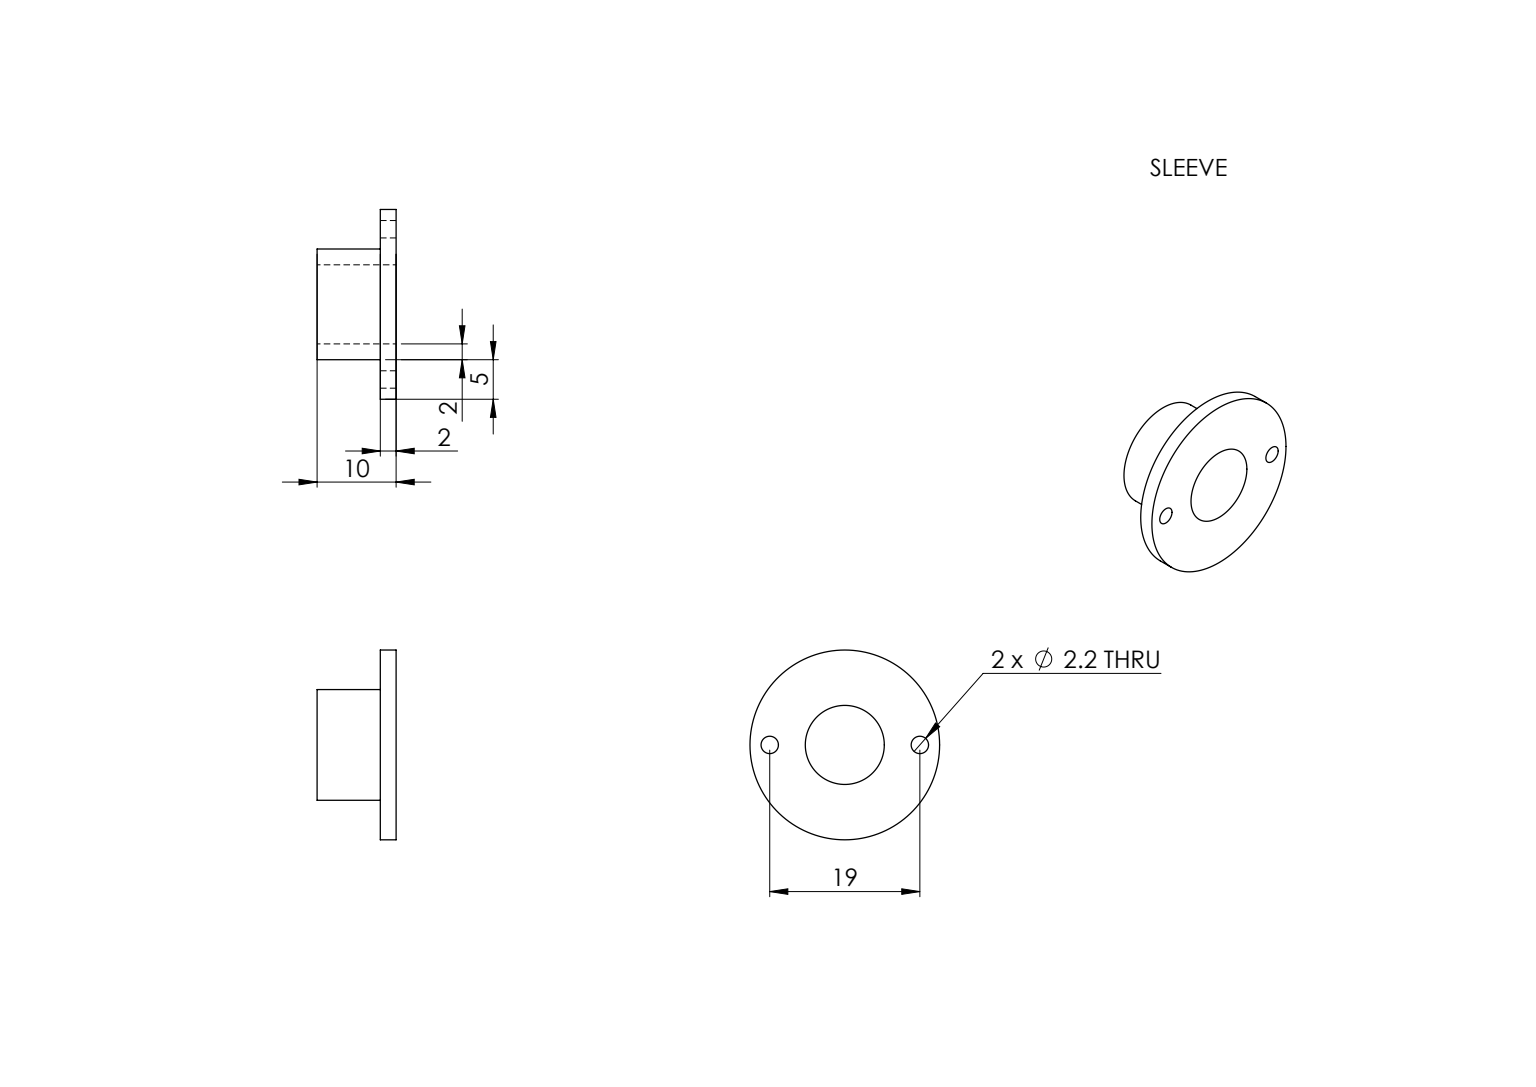
ISO-10303-21;
HEADER;
FILE_DESCRIPTION (('STEP AP214'),
    '1' );
FILE_NAME ('sleeve.step',
    '2026-10-27T14:18:53',
    ( '' ),
    ( '' ),
    'SwSTEP 2.0',
    'SolidWorks 2026',
    '' );
FILE_SCHEMA (( 'AUTOMOTIVE_DESIGN' ));
ENDSEC;

DATA;
#12=AXIS2_PLACEMENT_3D ( 'NONE', #3102, #281, #5829 ) ;
#16=AXIS2_PLACEMENT_3D ( 'NONE', #3293, #3357, #1408 ) ;
#82=DIRECTION ( 'NONE',  ( -1.000000000000000000, -0.000000000000000000, -0.000000000000000000 ) ) ;
#93=ADVANCED_FACE ( 'NONE', ( #1832 ), #5149, .T. ) ;
#96=AXIS2_PLACEMENT_3D ( 'NONE', #2644, #2066, #2156 ) ;
#106=EDGE_CURVE ( 'NONE', #5742, #4738, #1545, .T. ) ;
#119=VECTOR ( 'NONE', #946, 1000.000000000000000 ) ;
#134=CARTESIAN_POINT ( 'NONE',  ( 77.00000000000001421, 0.000000000000000000, -9.500000000000000000 ) ) ;
#163=DIRECTION ( 'NONE',  ( 1.000000000000000000, 0.000000000000000000, 0.000000000000000000 ) ) ;
#170=DIRECTION ( 'NONE',  ( 1.000000000000000000, 0.000000000000000000, 0.000000000000000000 ) ) ;
#184=EDGE_LOOP ( 'NONE', ( #1736, #1918, #2803, #4807 ) ) ;
#196=MANIFOLD_SOLID_BREP ( 'M2 Clearance Hole1', #4902 ) ;
#229=CYLINDRICAL_SURFACE ( 'NONE', #96, 5.000000000000000000 ) ;
#230=FACE_BOUND ( 'NONE', #460, .T. ) ;
#260=CARTESIAN_POINT ( 'NONE',  ( 67.00000000000001421, 6.123233995736766282E-16, 5.000000000000000000 ) ) ;
#281=DIRECTION ( 'NONE',  ( 1.000000000000000000, 0.000000000000000000, 0.000000000000000000 ) ) ;
#292=EDGE_LOOP ( 'NONE', ( #561, #1118, #3736, #5489 ) ) ;
#331=ORIENTED_EDGE ( 'NONE', *, *, #2483, .F. ) ;
#333=EDGE_CURVE ( 'NONE', #4738, #5742, #4095, .T. ) ;
#379=ORIENTED_EDGE ( 'NONE', *, *, #3057, .F. ) ;
#406=VECTOR ( 'NONE', #2782, 1000.000000000000000 ) ;
#435=AXIS2_PLACEMENT_3D ( 'NONE', #5878, #3224, #2274 ) ;
#460=EDGE_LOOP ( 'NONE', ( #331, #4146 ) ) ;
#464=DIRECTION ( 'NONE',  ( 0.000000000000000000, 0.000000000000000000, -1.000000000000000000 ) ) ;
#474=LINE ( 'NONE', #5100, #406 ) ;
#485=CARTESIAN_POINT ( 'NONE',  ( 77.00000000000001421, 0.000000000000000000, -9.500000000000000000 ) ) ;
#493=CIRCLE ( 'NONE', #4373, 1.099999999999998535 ) ;
#494=PRODUCT ( 'sleeve', 'sleeve', '', ( #2080 ) ) ;
#495=ORIENTED_EDGE ( 'NONE', *, *, #5762, .T. ) ;
#498=CIRCLE ( 'NONE', #1367, 1.099999999999998535 ) ;
#500=VERTEX_POINT ( 'NONE', #5168 ) ;
#502=VECTOR ( 'NONE', #1263, 1000.000000000000000 ) ;
#530=CARTESIAN_POINT ( 'NONE',  ( 77.00000000000001421, 0.000000000000000000, 0.000000000000000000 ) ) ;
#534=DIRECTION ( 'NONE',  ( 0.000000000000000000, 0.000000000000000000, -1.000000000000000000 ) ) ;
#545=DIRECTION ( 'NONE',  ( 0.000000000000000000, 0.000000000000000000, -1.000000000000000000 ) ) ;
#556=( LENGTH_UNIT ( ) NAMED_UNIT ( * ) SI_UNIT ( .MILLI., .METRE. ) );
#561=ORIENTED_EDGE ( 'NONE', *, *, #2602, .F. ) ;
#573=UNCERTAINTY_MEASURE_WITH_UNIT (LENGTH_MEASURE( 1.000000000000000082E-05 ), #1086, 'distance_accuracy_value', 'NONE');
#577=FACE_OUTER_BOUND ( 'NONE', #2183, .T. ) ;
#584=CARTESIAN_POINT ( 'NONE',  ( 67.00000000000001421, 0.000000000000000000, 0.000000000000000000 ) ) ;
#587=CIRCLE ( 'NONE', #1933, 1.099999999999998535 ) ;
#594=DIRECTION ( 'NONE',  ( 1.000000000000000000, -0.000000000000000000, -0.000000000000000000 ) ) ;
#597=AXIS2_PLACEMENT_3D ( 'NONE', #715, #5362, #4077 ) ;
#607=ORIENTED_EDGE ( 'NONE', *, *, #3154, .F. ) ;
#617=ADVANCED_FACE ( 'NONE', ( #2607 ), #229, .F. ) ;
#653=FACE_OUTER_BOUND ( 'NONE', #742, .T. ) ;
#661=DIRECTION ( 'NONE',  ( 1.000000000000000000, -0.000000000000000000, -0.000000000000000000 ) ) ;
#667=DIRECTION ( 'NONE',  ( 1.000000000000000000, 0.000000000000000000, 0.000000000000000000 ) ) ;
#698=VERTEX_POINT ( 'NONE', #4958 ) ;
#707=PLANE ( 'NONE',  #3487 ) ;
#715=CARTESIAN_POINT ( 'NONE',  ( 75.00000000000001421, 0.000000000000000000, 0.000000000000000000 ) ) ;
#742=EDGE_LOOP ( 'NONE', ( #3170, #5345, #1739, #1388 ) ) ;
#768=ORIENTED_EDGE ( 'NONE', *, *, #864, .F. ) ;
#793=EDGE_CURVE ( 'NONE', #853, #1083, #1370, .T. ) ;
#836=ORIENTED_EDGE ( 'NONE', *, *, #106, .F. ) ;
#853=VERTEX_POINT ( 'NONE', #1421 ) ;
#864=EDGE_CURVE ( 'NONE', #1686, #2079, #5088, .T. ) ;
#865=CIRCLE ( 'NONE', #5519, 7.000000000000000000 ) ;
#871=CIRCLE ( 'NONE', #1922, 5.000000000000000000 ) ;
#885=ORIENTED_EDGE ( 'NONE', *, *, #4953, .F. ) ;
#912=DIRECTION ( 'NONE',  ( 0.000000000000000000, 0.000000000000000000, -1.000000000000000000 ) ) ;
#940=DIRECTION ( 'NONE',  ( 1.000000000000000000, -0.000000000000000000, -0.000000000000000000 ) ) ;
#945=ADVANCED_FACE ( 'NONE', ( #1482 ), #1994, .F. ) ;
#946=DIRECTION ( 'NONE',  ( -1.000000000000000000, -0.000000000000000000, -0.000000000000000000 ) ) ;
#952=DIRECTION ( 'NONE',  ( 1.000000000000000000, 0.000000000000000000, 0.000000000000000000 ) ) ;
#986=CARTESIAN_POINT ( 'NONE',  ( 77.00000000000001421, 0.000000000000000000, 9.500000000000000000 ) ) ;
#1007=DIRECTION ( 'NONE',  ( 0.000000000000000000, 0.000000000000000000, -1.000000000000000000 ) ) ;
#1014=DIRECTION ( 'NONE',  ( 0.000000000000000000, 0.000000000000000000, -1.000000000000000000 ) ) ;
#1020=DIRECTION ( 'NONE',  ( 1.000000000000000000, 0.000000000000000000, 0.000000000000000000 ) ) ;
#1025=ORIENTED_EDGE ( 'NONE', *, *, #3057, .T. ) ;
#1033=VERTEX_POINT ( 'NONE', #5730 ) ;
#1039=CARTESIAN_POINT ( 'NONE',  ( 67.00000000000001421, 0.000000000000000000, -7.000000000000000000 ) ) ;
#1051=UNCERTAINTY_MEASURE_WITH_UNIT (LENGTH_MEASURE( 1.000000000000000082E-05 ), #556, 'distance_accuracy_value', 'NONE');
#1066=ORIENTED_EDGE ( 'NONE', *, *, #3945, .F. ) ;
#1075=CARTESIAN_POINT ( 'NONE',  ( 77.00000000000001421, 6.123233995736766282E-16, 5.000000000000000000 ) ) ;
#1079=VECTOR ( 'NONE', #4669, 1000.000000000000000 ) ;
#1083=VERTEX_POINT ( 'NONE', #2974 ) ;
#1086=( LENGTH_UNIT ( ) NAMED_UNIT ( * ) SI_UNIT ( .MILLI., .METRE. ) );
#1096=ORIENTED_EDGE ( 'NONE', *, *, #4928, .T. ) ;
#1097=EDGE_CURVE ( 'NONE', #698, #853, #5401, .T. ) ;
#1107=CARTESIAN_POINT ( 'NONE',  ( 67.00000000000001421, 0.000000000000000000, 0.000000000000000000 ) ) ;
#1118=ORIENTED_EDGE ( 'NONE', *, *, #4148, .T. ) ;
#1122=FACE_BOUND ( 'NONE', #4862, .T. ) ;
#1132=EDGE_LOOP ( 'NONE', ( #2391, #4516, #2697, #3573 ) ) ;
#1153=AXIS2_PLACEMENT_3D ( 'NONE', #1244, #5435, #4903 ) ;
#1174=EDGE_CURVE ( 'NONE', #3739, #3914, #1198, .T. ) ;
#1198=CIRCLE ( 'NONE', #435, 7.000000000000000000 ) ;
#1244=CARTESIAN_POINT ( 'NONE',  ( 77.00000000000001421, 0.000000000000000000, 0.000000000000000000 ) ) ;
#1247=ORIENTED_EDGE ( 'NONE', *, *, #2767, .F. ) ;
#1263=DIRECTION ( 'NONE',  ( 1.000000000000000000, -0.000000000000000000, -0.000000000000000000 ) ) ;
#1278=AXIS2_PLACEMENT_3D ( 'NONE', #5592, #2758, #4614 ) ;
#1300=ORIENTED_EDGE ( 'NONE', *, *, #2092, .T. ) ;
#1316=ORIENTED_EDGE ( 'NONE', *, *, #4317, .F. ) ;
#1328=LINE ( 'NONE', #3553, #3131 ) ;
#1351=CYLINDRICAL_SURFACE ( 'NONE', #1278, 1.099999999999998535 ) ;
#1359=PLANE ( 'NONE',  #4979 ) ;
#1367=AXIS2_PLACEMENT_3D ( 'NONE', #2010, #5780, #3474 ) ;
#1370=CIRCLE ( 'NONE', #3703, 1.099999999999998535 ) ;
#1371=FACE_BOUND ( 'NONE', #2481, .T. ) ;
#1388=ORIENTED_EDGE ( 'NONE', *, *, #793, .T. ) ;
#1396=ADVANCED_FACE ( 'NONE', ( #3274, #4676 ), #4731, .F. ) ;
#1408=DIRECTION ( 'NONE',  ( 0.000000000000000000, 0.000000000000000000, -1.000000000000000000 ) ) ;
#1421=CARTESIAN_POINT ( 'NONE',  ( 77.00000000000001421, 0.000000000000000000, -10.59999999999999787 ) ) ;
#1447=CARTESIAN_POINT ( 'NONE',  ( 75.00000000000001421, 0.000000000000000000, 9.500000000000000000 ) ) ;
#1453=EDGE_LOOP ( 'NONE', ( #836, #4145 ) ) ;
#1479=DIRECTION ( 'NONE',  ( 1.000000000000000000, 0.000000000000000000, 0.000000000000000000 ) ) ;
#1482=FACE_OUTER_BOUND ( 'NONE', #3024, .T. ) ;
#1487=CARTESIAN_POINT ( 'NONE',  ( 77.00000000000001421, 0.000000000000000000, 8.400000000000000355 ) ) ;
#1491=CARTESIAN_POINT ( 'NONE',  ( 77.00000000000001421, 0.000000000000000000, 0.000000000000000000 ) ) ;
#1496=CARTESIAN_POINT ( 'NONE',  ( 77.00000000000001421, 1.347111479062087271E-16, 10.59999999999999787 ) ) ;
#1509=EDGE_LOOP ( 'NONE', ( #4744, #2585 ) ) ;
#1524=VERTEX_POINT ( 'NONE', #1075 ) ;
#1544=ORIENTED_EDGE ( 'NONE', *, *, #1174, .T. ) ;
#1545=CIRCLE ( 'NONE', #4752, 12.00000000000000000 ) ;
#1554=CIRCLE ( 'NONE', #16, 5.000000000000000000 ) ;
#1566=CIRCLE ( 'NONE', #597, 7.000000000000000000 ) ;
#1596=ORIENTED_EDGE ( 'NONE', *, *, #2092, .F. ) ;
#1605=FILL_AREA_STYLE ('',( #2060 ) ) ;
#1610=EDGE_CURVE ( 'NONE', #3914, #3739, #4338, .T. ) ;
#1613=AXIS2_PLACEMENT_3D ( 'NONE', #2411, #1020, #5661 ) ;
#1621=DIRECTION ( 'NONE',  ( 1.000000000000000000, 0.000000000000000000, 0.000000000000000000 ) ) ;
#1625=CARTESIAN_POINT ( 'NONE',  ( 67.00000000000001421, 0.000000000000000000, -5.000000000000000000 ) ) ;
#1637=SURFACE_STYLE_USAGE ( .BOTH. , #5312 ) ;
#1686=VERTEX_POINT ( 'NONE', #3155 ) ;
#1700=CARTESIAN_POINT ( 'NONE',  ( 75.00000000000001421, 0.000000000000000000, 0.000000000000000000 ) ) ;
#1701=PRODUCT_DEFINITION_SHAPE ( 'NONE', 'NONE',  #2570 ) ;
#1726=DIRECTION ( 'NONE',  ( 1.000000000000000000, 0.000000000000000000, 0.000000000000000000 ) ) ;
#1736=ORIENTED_EDGE ( 'NONE', *, *, #2058, .F. ) ;
#1739=ORIENTED_EDGE ( 'NONE', *, *, #1097, .T. ) ;
#1745=AXIS2_PLACEMENT_3D ( 'NONE', #530, #82, #5327 ) ;
#1771=DIRECTION ( 'NONE',  ( 0.000000000000000000, 0.000000000000000000, -1.000000000000000000 ) ) ;
#1804=CARTESIAN_POINT ( 'NONE',  ( 75.00000000000001421, 0.000000000000000000, 0.000000000000000000 ) ) ;
#1810=CARTESIAN_POINT ( 'NONE',  ( 75.00000000000001421, 1.469576158976823947E-15, -12.00000000000000000 ) ) ;
#1813=VERTEX_POINT ( 'NONE', #1496 ) ;
#1832=FACE_OUTER_BOUND ( 'NONE', #292, .T. ) ;
#1833=AXIS2_PLACEMENT_3D ( 'NONE', #3894, #1621, #3443 ) ;
#1839=DIRECTION ( 'NONE',  ( 1.000000000000000000, -0.000000000000000000, -0.000000000000000000 ) ) ;
#1889=LINE ( 'NONE', #3356, #3200 ) ;
#1897=EDGE_CURVE ( 'NONE', #500, #1083, #1889, .T. ) ;
#1904=CARTESIAN_POINT ( 'NONE',  ( 67.00000000000001421, 0.000000000000000000, 0.000000000000000000 ) ) ;
#1913=( NAMED_UNIT ( * ) SI_UNIT ( $, .STERADIAN. ) SOLID_ANGLE_UNIT ( ) );
#1918=ORIENTED_EDGE ( 'NONE', *, *, #2276, .F. ) ;
#1922=AXIS2_PLACEMENT_3D ( 'NONE', #2652, #2830, #464 ) ;
#1933=AXIS2_PLACEMENT_3D ( 'NONE', #986, #2808, #4699 ) ;
#1942=ORIENTED_EDGE ( 'NONE', *, *, #2000, .T. ) ;
#1966=ORIENTED_EDGE ( 'NONE', *, *, #1097, .F. ) ;
#1978=CARTESIAN_POINT ( 'NONE',  ( 75.00000000000001421, 0.000000000000000000, 0.000000000000000000 ) ) ;
#1988=DIRECTION ( 'NONE',  ( 1.000000000000000000, 0.000000000000000000, 0.000000000000000000 ) ) ;
#1990=CARTESIAN_POINT ( 'NONE',  ( 77.00000000000001421, 0.000000000000000000, 9.500000000000000000 ) ) ;
#1994=CYLINDRICAL_SURFACE ( 'NONE', #5653, 5.000000000000000000 ) ;
#1995=ORIENTED_EDGE ( 'NONE', *, *, #2425, .T. ) ;
#2000=EDGE_CURVE ( 'NONE', #1524, #3408, #2315, .T. ) ;
#2010=CARTESIAN_POINT ( 'NONE',  ( 75.00000000000001421, 0.000000000000000000, -9.500000000000000000 ) ) ;
#2026=UNCERTAINTY_MEASURE_WITH_UNIT (LENGTH_MEASURE( 1.000000000000000082E-05 ), #2116, 'distance_accuracy_value', 'NONE');
#2058=EDGE_CURVE ( 'NONE', #5304, #1524, #2557, .T. ) ;
#2060=FILL_AREA_STYLE_COLOUR ( '', #2747 ) ;
#2066=DIRECTION ( 'NONE',  ( 1.000000000000000000, 0.000000000000000000, 0.000000000000000000 ) ) ;
#2079=VERTEX_POINT ( 'NONE', #5745 ) ;
#2080=PRODUCT_CONTEXT ( 'NONE', #5443, 'mechanical' ) ;
#2089=ORIENTED_EDGE ( 'NONE', *, *, #1610, .T. ) ;
#2092=EDGE_CURVE ( 'NONE', #2669, #4799, #865, .T. ) ;
#2098=EDGE_LOOP ( 'NONE', ( #3653, #1247, #495, #4762 ) ) ;
#2116=( LENGTH_UNIT ( ) NAMED_UNIT ( * ) SI_UNIT ( .MILLI., .METRE. ) );
#2123=VECTOR ( 'NONE', #170, 1000.000000000000000 ) ;
#2127=ORIENTED_EDGE ( 'NONE', *, *, #3252, .F. ) ;
#2135=AXIS2_PLACEMENT_3D ( 'NONE', #3768, #952, #1014 ) ;
#2156=DIRECTION ( 'NONE',  ( 0.000000000000000000, 0.000000000000000000, -1.000000000000000000 ) ) ;
#2164=PRODUCT_DEFINITION_FORMATION_WITH_SPECIFIED_SOURCE ( 'ANY', '', #494, .NOT_KNOWN. ) ;
#2183=EDGE_LOOP ( 'NONE', ( #3761, #5439, #4702, #1966 ) ) ;
#2227=CIRCLE ( 'NONE', #2423, 12.00000000000000000 ) ;
#2232=CARTESIAN_POINT ( 'NONE',  ( 67.00000000000001421, 0.000000000000000000, 0.000000000000000000 ) ) ;
#2237=CIRCLE ( 'NONE', #3780, 1.099999999999998535 ) ;
#2251=ORIENTED_EDGE ( 'NONE', *, *, #5010, .F. ) ;
#2257=MECHANICAL_DESIGN_GEOMETRIC_PRESENTATION_REPRESENTATION('',(#4595),#3711);
#2274=DIRECTION ( 'NONE',  ( 0.000000000000000000, 0.000000000000000000, -1.000000000000000000 ) ) ;
#2276=EDGE_CURVE ( 'NONE', #3852, #5304, #871, .T. ) ;
#2315=CIRCLE ( 'NONE', #1833, 5.000000000000000000 ) ;
#2321=AXIS2_PLACEMENT_3D ( 'NONE', #4119, #2350, #4083 ) ;
#2322=CARTESIAN_POINT ( 'NONE',  ( 77.00000000000001421, 0.000000000000000000, -9.500000000000000000 ) ) ;
#2323=CIRCLE ( 'NONE', #12, 5.000000000000000000 ) ;
#2330=DIRECTION ( 'NONE',  ( 1.000000000000000000, -0.000000000000000000, -0.000000000000000000 ) ) ;
#2338=CARTESIAN_POINT ( 'NONE',  ( 75.00000000000001421, 0.000000000000000000, 0.000000000000000000 ) ) ;
#2344=ADVANCED_FACE ( 'NONE', ( #1371, #1122, #2920, #230 ), #707, .T. ) ;
#2350=DIRECTION ( 'NONE',  ( -1.000000000000000000, -0.000000000000000000, -0.000000000000000000 ) ) ;
#2362=VECTOR ( 'NONE', #4861, 1000.000000000000000 ) ;
#2366=DIRECTION ( 'NONE',  ( 0.000000000000000000, 0.000000000000000000, -1.000000000000000000 ) ) ;
#2391=ORIENTED_EDGE ( 'NONE', *, *, #3208, .F. ) ;
#2411=CARTESIAN_POINT ( 'NONE',  ( 67.00000000000001421, 0.000000000000000000, 0.000000000000000000 ) ) ;
#2423=AXIS2_PLACEMENT_3D ( 'NONE', #4705, #1988, #2874 ) ;
#2425=EDGE_CURVE ( 'NONE', #500, #698, #2610, .T. ) ;
#2429=CYLINDRICAL_SURFACE ( 'NONE', #4096, 1.099999999999998535 ) ;
#2438=AXIS2_PLACEMENT_3D ( 'NONE', #584, #5675, #1007 ) ;
#2462=CARTESIAN_POINT ( 'NONE',  ( 75.00000000000001421, 0.000000000000000000, -9.500000000000000000 ) ) ;
#2463=ORIENTED_EDGE ( 'NONE', *, *, #4160, .F. ) ;
#2481=EDGE_LOOP ( 'NONE', ( #379, #2127 ) ) ;
#2482=AXIS2_PLACEMENT_3D ( 'NONE', #1107, #5754, #4337 ) ;
#2483=EDGE_CURVE ( 'NONE', #3408, #1524, #2323, .T. ) ;
#2513=MECHANICAL_DESIGN_GEOMETRIC_PRESENTATION_REPRESENTATION('',(#5058),#3689);
#2552=DIRECTION ( 'NONE',  ( 0.000000000000000000, 0.000000000000000000, -1.000000000000000000 ) ) ;
#2557=LINE ( 'NONE', #260, #2123 ) ;
#2570=PRODUCT_DEFINITION ( 'UNKNOWN', '', #2164, #5792 ) ;
#2574=( NAMED_UNIT ( * ) SI_UNIT ( $, .STERADIAN. ) SOLID_ANGLE_UNIT ( ) );
#2585=ORIENTED_EDGE ( 'NONE', *, *, #1610, .F. ) ;
#2596=CARTESIAN_POINT ( 'NONE',  ( 77.00000000000001421, 0.000000000000000000, 8.400000000000000355 ) ) ;
#2602=EDGE_CURVE ( 'NONE', #5213, #1033, #2614, .T. ) ;
#2607=FACE_OUTER_BOUND ( 'NONE', #184, .T. ) ;
#2610=CIRCLE ( 'NONE', #4169, 1.099999999999998535 ) ;
#2614=CIRCLE ( 'NONE', #1153, 12.00000000000000000 ) ;
#2644=CARTESIAN_POINT ( 'NONE',  ( 67.00000000000001421, 0.000000000000000000, 0.000000000000000000 ) ) ;
#2647=( GEOMETRIC_REPRESENTATION_CONTEXT ( 3 ) GLOBAL_UNCERTAINTY_ASSIGNED_CONTEXT ( ( #2026 ) ) GLOBAL_UNIT_ASSIGNED_CONTEXT ( ( #2116, #5374, #4344 ) ) REPRESENTATION_CONTEXT ( 'NONE', 'WORKASPACE' ) );
#2652=CARTESIAN_POINT ( 'NONE',  ( 67.00000000000001421, 0.000000000000000000, 0.000000000000000000 ) ) ;
#2669=VERTEX_POINT ( 'NONE', #3811 ) ;
#2670=DIRECTION ( 'NONE',  ( 1.000000000000000000, -0.000000000000000000, -0.000000000000000000 ) ) ;
#2697=ORIENTED_EDGE ( 'NONE', *, *, #3252, .T. ) ;
#2703=ORIENTED_EDGE ( 'NONE', *, *, #2602, .T. ) ;
#2747=COLOUR_RGB ( '',0.8941176470588234615, 0.8941176470588234615, 0.8941176470588234615 ) ;
#2758=DIRECTION ( 'NONE',  ( 1.000000000000000000, -0.000000000000000000, -0.000000000000000000 ) ) ;
#2767=EDGE_CURVE ( 'NONE', #1033, #5213, #2227, .T. ) ;
#2782=DIRECTION ( 'NONE',  ( 1.000000000000000000, 0.000000000000000000, 0.000000000000000000 ) ) ;
#2795=DIRECTION ( 'NONE',  ( 0.000000000000000000, 0.000000000000000000, -1.000000000000000000 ) ) ;
#2801=LINE ( 'NONE', #4144, #3506 ) ;
#2803=ORIENTED_EDGE ( 'NONE', *, *, #5010, .T. ) ;
#2808=DIRECTION ( 'NONE',  ( 1.000000000000000000, -0.000000000000000000, -0.000000000000000000 ) ) ;
#2830=DIRECTION ( 'NONE',  ( 1.000000000000000000, 0.000000000000000000, 0.000000000000000000 ) ) ;
#2840=ADVANCED_FACE ( 'NONE', ( #577 ), #2429, .F. ) ;
#2874=DIRECTION ( 'NONE',  ( 0.000000000000000000, 0.000000000000000000, -1.000000000000000000 ) ) ;
#2907=DIRECTION ( 'NONE',  ( 0.000000000000000000, 0.000000000000000000, -1.000000000000000000 ) ) ;
#2920=FACE_OUTER_BOUND ( 'NONE', #5697, .T. ) ;
#2941=FACE_OUTER_BOUND ( 'NONE', #3622, .T. ) ;
#2974=CARTESIAN_POINT ( 'NONE',  ( 77.00000000000001421, 1.347111479062087271E-16, -8.400000000000000355 ) ) ;
#3024=EDGE_LOOP ( 'NONE', ( #607, #3147, #1942, #2251 ) ) ;
#3037=( NAMED_UNIT ( * ) PLANE_ANGLE_UNIT ( ) SI_UNIT ( $, .RADIAN. ) );
#3057=EDGE_CURVE ( 'NONE', #5651, #1813, #493, .T. ) ;
#3062=DIRECTION ( 'NONE',  ( 0.000000000000000000, 0.000000000000000000, -1.000000000000000000 ) ) ;
#3102=CARTESIAN_POINT ( 'NONE',  ( 77.00000000000001421, 0.000000000000000000, 0.000000000000000000 ) ) ;
#3105=ORIENTED_EDGE ( 'NONE', *, *, #3154, .T. ) ;
#3122=FACE_OUTER_BOUND ( 'NONE', #4657, .T. ) ;
#3131=VECTOR ( 'NONE', #2670, 1000.000000000000000 ) ;
#3133=DIRECTION ( 'NONE',  ( 0.000000000000000000, 0.000000000000000000, -1.000000000000000000 ) ) ;
#3147=ORIENTED_EDGE ( 'NONE', *, *, #2058, .T. ) ;
#3154=EDGE_CURVE ( 'NONE', #5304, #3852, #1554, .T. ) ;
#3155=CARTESIAN_POINT ( 'NONE',  ( 75.00000000000001421, 0.000000000000000000, 8.400000000000000355 ) ) ;
#3163=FACE_BOUND ( 'NONE', #5469, .T. ) ;
#3170=ORIENTED_EDGE ( 'NONE', *, *, #1897, .F. ) ;
#3200=VECTOR ( 'NONE', #4178, 1000.000000000000000 ) ;
#3208=EDGE_CURVE ( 'NONE', #2079, #1686, #3690, .T. ) ;
#3224=DIRECTION ( 'NONE',  ( 1.000000000000000000, 0.000000000000000000, 0.000000000000000000 ) ) ;
#3252=EDGE_CURVE ( 'NONE', #1813, #5651, #587, .T. ) ;
#3254=SHAPE_REPRESENTATION ( 'sleeve', ( #5080 ), #2647 ) ;
#3259=ADVANCED_FACE ( 'NONE', ( #4213 ), #5591, .T. ) ;
#3274=FACE_BOUND ( 'NONE', #4241, .T. ) ;
#3293=CARTESIAN_POINT ( 'NONE',  ( 67.00000000000001421, 0.000000000000000000, 0.000000000000000000 ) ) ;
#3297=CARTESIAN_POINT ( 'NONE',  ( 67.00000000000001421, 0.000000000000000000, -5.000000000000000000 ) ) ;
#3299=ORIENTED_EDGE ( 'NONE', *, *, #3945, .T. ) ;
#3308=DIRECTION ( 'NONE',  ( 1.000000000000000000, 0.000000000000000000, 0.000000000000000000 ) ) ;
#3331=LINE ( 'NONE', #5179, #1079 ) ;
#3348=CYLINDRICAL_SURFACE ( 'NONE', #2438, 7.000000000000000000 ) ;
#3356=CARTESIAN_POINT ( 'NONE',  ( 77.00000000000001421, 1.347111479062087271E-16, -8.400000000000000355 ) ) ;
#3357=DIRECTION ( 'NONE',  ( 1.000000000000000000, 0.000000000000000000, 0.000000000000000000 ) ) ;
#3369=DIRECTION ( 'NONE',  ( 1.000000000000000000, 0.000000000000000000, 0.000000000000000000 ) ) ;
#3408=VERTEX_POINT ( 'NONE', #4539 ) ;
#3413=DIRECTION ( 'NONE',  ( 1.000000000000000000, 0.000000000000000000, 0.000000000000000000 ) ) ;
#3443=DIRECTION ( 'NONE',  ( 0.000000000000000000, 0.000000000000000000, -1.000000000000000000 ) ) ;
#3458=SURFACE_STYLE_FILL_AREA ( #1605 ) ;
#3474=DIRECTION ( 'NONE',  ( 0.000000000000000000, 0.000000000000000000, -1.000000000000000000 ) ) ;
#3487=AXIS2_PLACEMENT_3D ( 'NONE', #1491, #3917, #2552 ) ;
#3506=VECTOR ( 'NONE', #1479, 1000.000000000000000 ) ;
#3527=CARTESIAN_POINT ( 'NONE',  ( 0.000000000000000000, 0.000000000000000000, 0.000000000000000000 ) ) ;
#3540=CARTESIAN_POINT ( 'NONE',  ( 67.00000000000001421, 6.123233995736766282E-16, 5.000000000000000000 ) ) ;
#3547=DIRECTION ( 'NONE',  ( 1.000000000000000000, 0.000000000000000000, 0.000000000000000000 ) ) ;
#3553=CARTESIAN_POINT ( 'NONE',  ( 77.00000000000001421, 1.347111479062087271E-16, 10.59999999999999787 ) ) ;
#3573=ORIENTED_EDGE ( 'NONE', *, *, #5640, .F. ) ;
#3579=APPLICATION_CONTEXT ( 'automotive_design' ) ;
#3622=EDGE_LOOP ( 'NONE', ( #1316, #768, #4153, #1025 ) ) ;
#3653=ORIENTED_EDGE ( 'NONE', *, *, #4148, .F. ) ;
#3689=( GEOMETRIC_REPRESENTATION_CONTEXT ( 3 ) GLOBAL_UNCERTAINTY_ASSIGNED_CONTEXT ( ( #1051 ) ) GLOBAL_UNIT_ASSIGNED_CONTEXT ( ( #556, #4235, #1913 ) ) REPRESENTATION_CONTEXT ( 'NONE', 'WORKASPACE' ) );
#3690=CIRCLE ( 'NONE', #2135, 1.099999999999998535 ) ;
#3703=AXIS2_PLACEMENT_3D ( 'NONE', #485, #2330, #912 ) ;
#3711=( GEOMETRIC_REPRESENTATION_CONTEXT ( 3 ) GLOBAL_UNCERTAINTY_ASSIGNED_CONTEXT ( ( #573 ) ) GLOBAL_UNIT_ASSIGNED_CONTEXT ( ( #1086, #3037, #2574 ) ) REPRESENTATION_CONTEXT ( 'NONE', 'WORKASPACE' ) );
#3716=AXIS2_PLACEMENT_3D ( 'NONE', #1447, #3369, #545 ) ;
#3736=ORIENTED_EDGE ( 'NONE', *, *, #333, .T. ) ;
#3739=VERTEX_POINT ( 'NONE', #1039 ) ;
#3761=ORIENTED_EDGE ( 'NONE', *, *, #2425, .F. ) ;
#3768=CARTESIAN_POINT ( 'NONE',  ( 75.00000000000001421, 0.000000000000000000, 9.500000000000000000 ) ) ;
#3780=AXIS2_PLACEMENT_3D ( 'NONE', #2322, #1839, #534 ) ;
#3811=CARTESIAN_POINT ( 'NONE',  ( 75.00000000000001421, 8.572527594031473190E-16, 7.000000000000000000 ) ) ;
#3832=DIRECTION ( 'NONE',  ( 0.000000000000000000, 0.000000000000000000, -1.000000000000000000 ) ) ;
#3842=ORIENTED_EDGE ( 'NONE', *, *, #793, .F. ) ;
#3844=SHAPE_REPRESENTATION_RELATIONSHIP ( 'NONE' , 'NONE' ,  #3254, #4722 ) ;
#3852=VERTEX_POINT ( 'NONE', #1625 ) ;
#3874=EDGE_LOOP ( 'NONE', ( #4834, #5576 ) ) ;
#3894=CARTESIAN_POINT ( 'NONE',  ( 77.00000000000001421, 0.000000000000000000, 0.000000000000000000 ) ) ;
#3914=VERTEX_POINT ( 'NONE', #5865 ) ;
#3917=DIRECTION ( 'NONE',  ( 1.000000000000000000, 0.000000000000000000, 0.000000000000000000 ) ) ;
#3945=EDGE_CURVE ( 'NONE', #4799, #2669, #1566, .T. ) ;
#3971=FACE_BOUND ( 'NONE', #4878, .T. ) ;
#4069=ORIENTED_EDGE ( 'NONE', *, *, #4160, .T. ) ;
#4077=DIRECTION ( 'NONE',  ( 0.000000000000000000, 0.000000000000000000, -1.000000000000000000 ) ) ;
#4083=DIRECTION ( 'NONE',  ( 0.000000000000000000, 0.000000000000000000, 1.000000000000000000 ) ) ;
#4088=CYLINDRICAL_SURFACE ( 'NONE', #5077, 7.000000000000000000 ) ;
#4095=CIRCLE ( 'NONE', #4201, 12.00000000000000000 ) ;
#4096=AXIS2_PLACEMENT_3D ( 'NONE', #134, #940, #2795 ) ;
#4119=CARTESIAN_POINT ( 'NONE',  ( 77.00000000000001421, 0.000000000000000000, 0.000000000000000000 ) ) ;
#4122=DIRECTION ( 'NONE',  ( 0.000000000000000000, 0.000000000000000000, -1.000000000000000000 ) ) ;
#4144=CARTESIAN_POINT ( 'NONE',  ( 67.00000000000001421, 8.572527594031473190E-16, 7.000000000000000000 ) ) ;
#4145=ORIENTED_EDGE ( 'NONE', *, *, #333, .F. ) ;
#4146=ORIENTED_EDGE ( 'NONE', *, *, #2000, .F. ) ;
#4148=EDGE_CURVE ( 'NONE', #5213, #4738, #5117, .T. ) ;
#4153=ORIENTED_EDGE ( 'NONE', *, *, #5640, .T. ) ;
#4160=EDGE_CURVE ( 'NONE', #3914, #2669, #2801, .T. ) ;
#4169=AXIS2_PLACEMENT_3D ( 'NONE', #2462, #163, #5320 ) ;
#4178=DIRECTION ( 'NONE',  ( 1.000000000000000000, -0.000000000000000000, -0.000000000000000000 ) ) ;
#4182=CARTESIAN_POINT ( 'NONE',  ( 75.00000000000001421, 0.000000000000000000, 12.00000000000000000 ) ) ;
#4201=AXIS2_PLACEMENT_3D ( 'NONE', #2338, #5922, #1771 ) ;
#4213=FACE_OUTER_BOUND ( 'NONE', #2098, .T. ) ;
#4226=ADVANCED_FACE ( 'NONE', ( #4440 ), #3348, .T. ) ;
#4235=( NAMED_UNIT ( * ) PLANE_ANGLE_UNIT ( ) SI_UNIT ( $, .RADIAN. ) );
#4240=LINE ( 'NONE', #3297, #5245 ) ;
#4241=EDGE_LOOP ( 'NONE', ( #5233, #3105 ) ) ;
#4257=ADVANCED_FACE ( 'NONE', ( #5463, #3163, #4991, #3971 ), #1359, .F. ) ;
#4304=CARTESIAN_POINT ( 'NONE',  ( 77.00000000000001421, 0.000000000000000000, -9.500000000000000000 ) ) ;
#4317=EDGE_CURVE ( 'NONE', #2079, #1813, #1328, .T. ) ;
#4337=DIRECTION ( 'NONE',  ( 0.000000000000000000, 0.000000000000000000, -1.000000000000000000 ) ) ;
#4338=CIRCLE ( 'NONE', #2482, 7.000000000000000000 ) ;
#4344=( NAMED_UNIT ( * ) SI_UNIT ( $, .STERADIAN. ) SOLID_ANGLE_UNIT ( ) );
#4373=AXIS2_PLACEMENT_3D ( 'NONE', #5872, #5513, #4122 ) ;
#4380=AXIS2_PLACEMENT_3D ( 'NONE', #4304, #594, #3832 ) ;
#4440=FACE_OUTER_BOUND ( 'NONE', #5734, .T. ) ;
#4516=ORIENTED_EDGE ( 'NONE', *, *, #4317, .T. ) ;
#4539=CARTESIAN_POINT ( 'NONE',  ( 77.00000000000001421, 0.000000000000000000, -5.000000000000000000 ) ) ;
#4595=STYLED_ITEM ( 'NONE', ( #5248 ), #4722 ) ;
#4614=DIRECTION ( 'NONE',  ( 0.000000000000000000, 0.000000000000000000, -1.000000000000000000 ) ) ;
#4637=FACE_OUTER_BOUND ( 'NONE', #1132, .T. ) ;
#4657=EDGE_LOOP ( 'NONE', ( #2463, #2089, #1096, #1596 ) ) ;
#4669=DIRECTION ( 'NONE',  ( -1.000000000000000000, -0.000000000000000000, -0.000000000000000000 ) ) ;
#4676=FACE_OUTER_BOUND ( 'NONE', #1509, .T. ) ;
#4693=ADVANCED_FACE ( 'NONE', ( #2941 ), #5371, .F. ) ;
#4699=DIRECTION ( 'NONE',  ( 0.000000000000000000, 0.000000000000000000, -1.000000000000000000 ) ) ;
#4702=ORIENTED_EDGE ( 'NONE', *, *, #4953, .T. ) ;
#4705=CARTESIAN_POINT ( 'NONE',  ( 77.00000000000001421, 0.000000000000000000, 0.000000000000000000 ) ) ;
#4722=ADVANCED_BREP_SHAPE_REPRESENTATION ( '', ( #196, #5080 ), #2647 ) ;
#4731=PLANE ( 'NONE',  #1613 ) ;
#4738=VERTEX_POINT ( 'NONE', #1810 ) ;
#4744=ORIENTED_EDGE ( 'NONE', *, *, #1174, .F. ) ;
#4752=AXIS2_PLACEMENT_3D ( 'NONE', #1804, #5933, #5037 ) ;
#4756=SHAPE_DEFINITION_REPRESENTATION ( #1701, #3254 ) ;
#4762=ORIENTED_EDGE ( 'NONE', *, *, #106, .T. ) ;
#4799=VERTEX_POINT ( 'NONE', #5970 ) ;
#4807=ORIENTED_EDGE ( 'NONE', *, *, #2483, .T. ) ;
#4808=ORIENTED_EDGE ( 'NONE', *, *, #4928, .F. ) ;
#4831=DIRECTION ( 'NONE',  ( 0.000000000000000000, 0.000000000000000000, 1.000000000000000000 ) ) ;
#4834=ORIENTED_EDGE ( 'NONE', *, *, #864, .T. ) ;
#4861=DIRECTION ( 'NONE',  ( 1.000000000000000000, -0.000000000000000000, -0.000000000000000000 ) ) ;
#4862=EDGE_LOOP ( 'NONE', ( #3842, #885 ) ) ;
#4878=EDGE_LOOP ( 'NONE', ( #3299, #1300 ) ) ;
#4902=CLOSED_SHELL ( 'NONE', ( #5695, #2840, #945, #4226, #93, #2344, #4257, #3259, #5582, #1396, #617, #5169, #4693 ) ) ;
#4903=DIRECTION ( 'NONE',  ( 0.000000000000000000, 0.000000000000000000, -1.000000000000000000 ) ) ;
#4928=EDGE_CURVE ( 'NONE', #3739, #4799, #474, .T. ) ;
#4953=EDGE_CURVE ( 'NONE', #1083, #853, #2237, .T. ) ;
#4958=CARTESIAN_POINT ( 'NONE',  ( 75.00000000000001421, 0.000000000000000000, -10.59999999999999787 ) ) ;
#4979=AXIS2_PLACEMENT_3D ( 'NONE', #1700, #1726, #3133 ) ;
#4983=LINE ( 'NONE', #2596, #502 ) ;
#4991=FACE_OUTER_BOUND ( 'NONE', #1453, .T. ) ;
#5010=EDGE_CURVE ( 'NONE', #3852, #3408, #4240, .T. ) ;
#5037=DIRECTION ( 'NONE',  ( 0.000000000000000000, 0.000000000000000000, -1.000000000000000000 ) ) ;
#5058=STYLED_ITEM('',(#6006),#196);
#5064=AXIS2_PLACEMENT_3D ( 'NONE', #1990, #661, #2907 ) ;
#5077=AXIS2_PLACEMENT_3D ( 'NONE', #2232, #3547, #3062 ) ;
#5080=AXIS2_PLACEMENT_3D ( 'NONE', #3527, #4831, #667 ) ;
#5088=CIRCLE ( 'NONE', #3716, 1.099999999999998535 ) ;
#5100=CARTESIAN_POINT ( 'NONE',  ( 67.00000000000001421, 0.000000000000000000, -7.000000000000000000 ) ) ;
#5109=EDGE_CURVE ( 'NONE', #698, #500, #498, .T. ) ;
#5117=LINE ( 'NONE', #5561, #119 ) ;
#5149=CYLINDRICAL_SURFACE ( 'NONE', #2321, 12.00000000000000000 ) ;
#5168=CARTESIAN_POINT ( 'NONE',  ( 75.00000000000001421, 1.347111479062087764E-16, -8.400000000000000355 ) ) ;
#5169=ADVANCED_FACE ( 'NONE', ( #653 ), #5231, .F. ) ;
#5179=CARTESIAN_POINT ( 'NONE',  ( 77.00000000000001421, 0.000000000000000000, 12.00000000000000000 ) ) ;
#5213=VERTEX_POINT ( 'NONE', #5843 ) ;
#5223=ORIENTED_EDGE ( 'NONE', *, *, #2767, .T. ) ;
#5231=CYLINDRICAL_SURFACE ( 'NONE', #4380, 1.099999999999998535 ) ;
#5233=ORIENTED_EDGE ( 'NONE', *, *, #2276, .T. ) ;
#5245=VECTOR ( 'NONE', #5593, 1000.000000000000000 ) ;
#5248=PRESENTATION_STYLE_ASSIGNMENT (( #1637 ) ) ;
#5297=DIRECTION ( 'NONE',  ( 0.000000000000000000, 0.000000000000000000, -1.000000000000000000 ) ) ;
#5304=VERTEX_POINT ( 'NONE', #3540 ) ;
#5312=SURFACE_SIDE_STYLE ('',( #3458 ) ) ;
#5320=DIRECTION ( 'NONE',  ( 0.000000000000000000, 0.000000000000000000, -1.000000000000000000 ) ) ;
#5327=DIRECTION ( 'NONE',  ( 0.000000000000000000, 0.000000000000000000, 1.000000000000000000 ) ) ;
#5344=CARTESIAN_POINT ( 'NONE',  ( 77.00000000000001421, 0.000000000000000000, -10.59999999999999787 ) ) ;
#5345=ORIENTED_EDGE ( 'NONE', *, *, #5109, .F. ) ;
#5362=DIRECTION ( 'NONE',  ( 1.000000000000000000, 0.000000000000000000, 0.000000000000000000 ) ) ;
#5371=CYLINDRICAL_SURFACE ( 'NONE', #5064, 1.099999999999998535 ) ;
#5374=( NAMED_UNIT ( * ) PLANE_ANGLE_UNIT ( ) SI_UNIT ( $, .RADIAN. ) );
#5401=LINE ( 'NONE', #5344, #2362 ) ;
#5435=DIRECTION ( 'NONE',  ( 1.000000000000000000, 0.000000000000000000, 0.000000000000000000 ) ) ;
#5439=ORIENTED_EDGE ( 'NONE', *, *, #1897, .T. ) ;
#5443=APPLICATION_CONTEXT ( 'automotive_design' ) ;
#5463=FACE_BOUND ( 'NONE', #3874, .T. ) ;
#5469=EDGE_LOOP ( 'NONE', ( #5658, #1995 ) ) ;
#5489=ORIENTED_EDGE ( 'NONE', *, *, #5762, .F. ) ;
#5513=DIRECTION ( 'NONE',  ( 1.000000000000000000, -0.000000000000000000, -0.000000000000000000 ) ) ;
#5519=AXIS2_PLACEMENT_3D ( 'NONE', #1978, #3413, #5297 ) ;
#5561=CARTESIAN_POINT ( 'NONE',  ( 77.00000000000001421, 1.469576158976823947E-15, -12.00000000000000000 ) ) ;
#5576=ORIENTED_EDGE ( 'NONE', *, *, #3208, .T. ) ;
#5582=ADVANCED_FACE ( 'NONE', ( #3122 ), #4088, .T. ) ;
#5591=CYLINDRICAL_SURFACE ( 'NONE', #1745, 12.00000000000000000 ) ;
#5592=CARTESIAN_POINT ( 'NONE',  ( 77.00000000000001421, 0.000000000000000000, 9.500000000000000000 ) ) ;
#5593=DIRECTION ( 'NONE',  ( 1.000000000000000000, 0.000000000000000000, 0.000000000000000000 ) ) ;
#5640=EDGE_CURVE ( 'NONE', #1686, #5651, #4983, .T. ) ;
#5651=VERTEX_POINT ( 'NONE', #1487 ) ;
#5653=AXIS2_PLACEMENT_3D ( 'NONE', #1904, #3308, #2366 ) ;
#5658=ORIENTED_EDGE ( 'NONE', *, *, #5109, .T. ) ;
#5661=DIRECTION ( 'NONE',  ( 0.000000000000000000, 0.000000000000000000, -1.000000000000000000 ) ) ;
#5675=DIRECTION ( 'NONE',  ( 1.000000000000000000, 0.000000000000000000, 0.000000000000000000 ) ) ;
#5695=ADVANCED_FACE ( 'NONE', ( #4637 ), #1351, .F. ) ;
#5697=EDGE_LOOP ( 'NONE', ( #5223, #2703 ) ) ;
#5730=CARTESIAN_POINT ( 'NONE',  ( 77.00000000000001421, 0.000000000000000000, 12.00000000000000000 ) ) ;
#5734=EDGE_LOOP ( 'NONE', ( #1544, #4069, #1066, #4808 ) ) ;
#5742=VERTEX_POINT ( 'NONE', #4182 ) ;
#5745=CARTESIAN_POINT ( 'NONE',  ( 75.00000000000001421, 1.347111479062087764E-16, 10.59999999999999787 ) ) ;
#5754=DIRECTION ( 'NONE',  ( 1.000000000000000000, 0.000000000000000000, 0.000000000000000000 ) ) ;
#5762=EDGE_CURVE ( 'NONE', #1033, #5742, #3331, .T. ) ;
#5780=DIRECTION ( 'NONE',  ( 1.000000000000000000, 0.000000000000000000, 0.000000000000000000 ) ) ;
#5792=PRODUCT_DEFINITION_CONTEXT ( 'detailed design', #3579, 'design' ) ;
#5829=DIRECTION ( 'NONE',  ( 0.000000000000000000, 0.000000000000000000, -1.000000000000000000 ) ) ;
#5843=CARTESIAN_POINT ( 'NONE',  ( 77.00000000000001421, 1.469576158976823947E-15, -12.00000000000000000 ) ) ;
#5865=CARTESIAN_POINT ( 'NONE',  ( 67.00000000000001421, 8.572527594031473190E-16, 7.000000000000000000 ) ) ;
#5872=CARTESIAN_POINT ( 'NONE',  ( 77.00000000000001421, 0.000000000000000000, 9.500000000000000000 ) ) ;
#5878=CARTESIAN_POINT ( 'NONE',  ( 67.00000000000001421, 0.000000000000000000, 0.000000000000000000 ) ) ;
#5922=DIRECTION ( 'NONE',  ( 1.000000000000000000, 0.000000000000000000, 0.000000000000000000 ) ) ;
#5933=DIRECTION ( 'NONE',  ( 1.000000000000000000, 0.000000000000000000, 0.000000000000000000 ) ) ;
#5970=CARTESIAN_POINT ( 'NONE',  ( 75.00000000000001421, 0.000000000000000000, -7.000000000000000000 ) ) ;
#6000=COLOUR_RGB('Light Blue',0.38,0.62,0.78);
#6001=FILL_AREA_STYLE_COLOUR('',#6000);
#6002=FILL_AREA_STYLE('',(#6001));
#6003=SURFACE_STYLE_FILL_AREA(#6002);
#6004=SURFACE_SIDE_STYLE('',(#6003));
#6005=SURFACE_STYLE_USAGE(.BOTH.,#6004);
#6006=PRESENTATION_STYLE_ASSIGNMENT((#6005));
ENDSEC;
END-ISO-10303-21;
